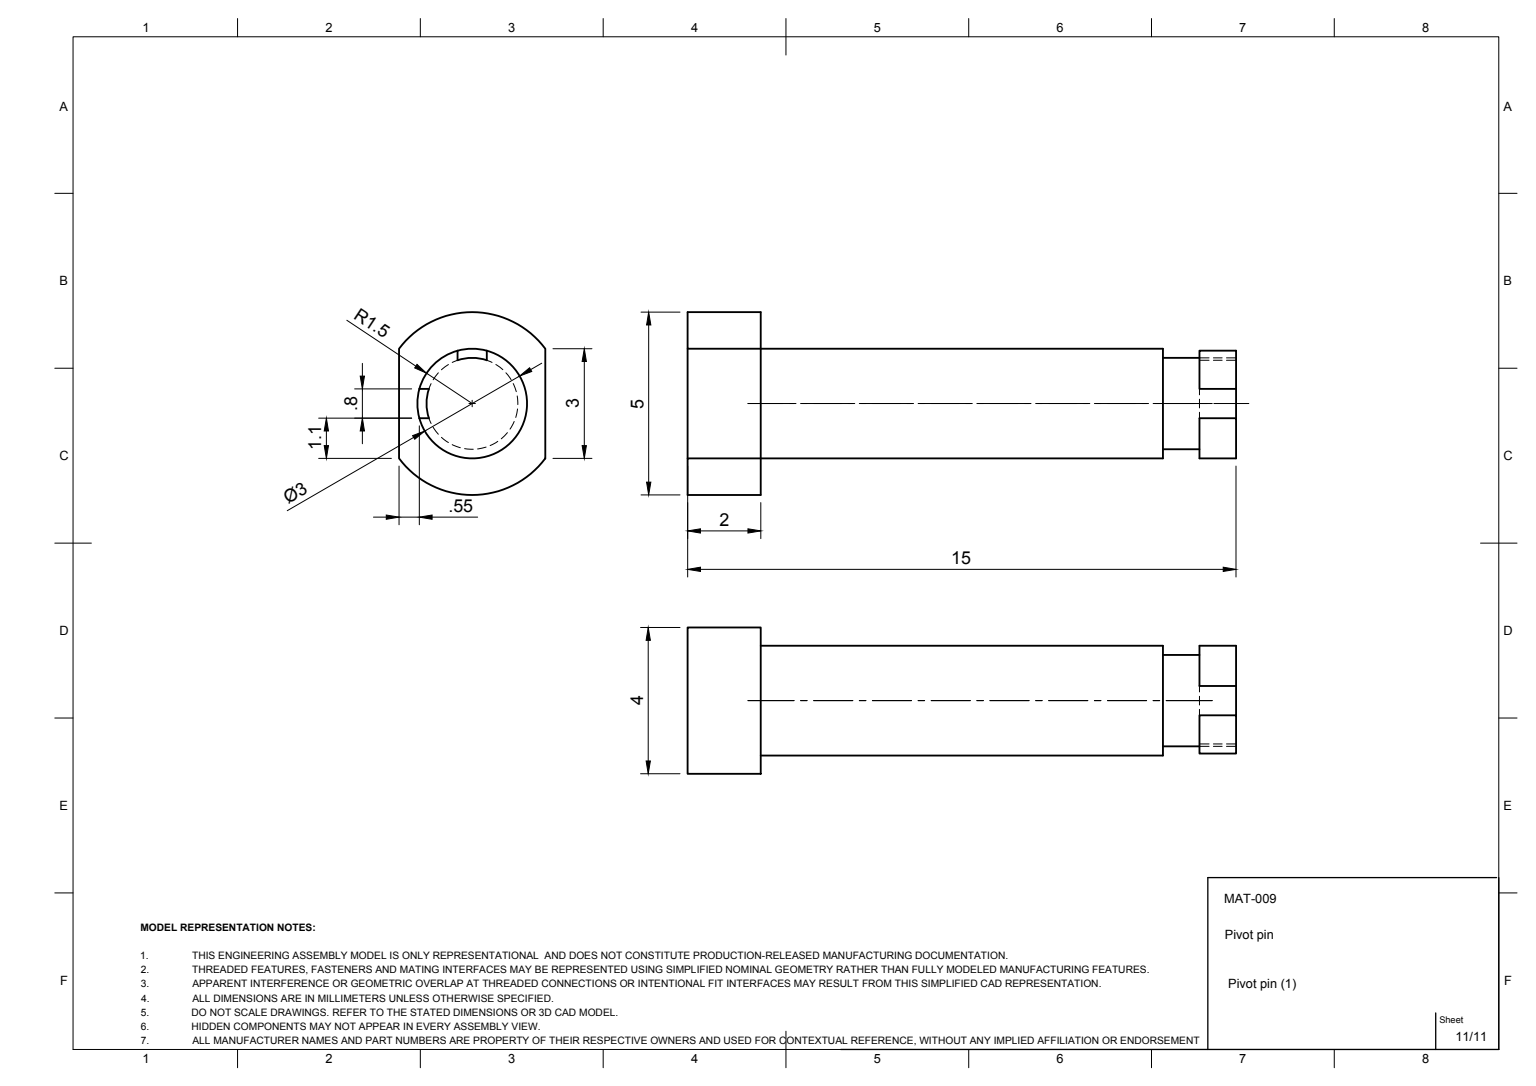
ISO-10303-21;
HEADER;
/* Generated by software containing ST-Developer
 * from STEP Tools, Inc. (www.steptools.com) 
 */

FILE_DESCRIPTION(
/* description */ ('STEP AP214'),
/* implementation_level */ '2;1');

FILE_NAME(
/* name */ 'Pivot Pin.step',
/* time_stamp */ '2026-11-14T05:43:09-08:00',
/* author */ (''),
/* organization */ (''),
/* preprocessor_version */ 'ST-DEVELOPER v20.2',
/* originating_system */ 'Autodesk Translation Framework v15.17.0.0',
/* authorisation */ '');

FILE_SCHEMA (('AUTOMOTIVE_DESIGN { 1 0 10303 214 3 1 1 }'));
ENDSEC;

DATA;
#10=MECHANICAL_DESIGN_GEOMETRIC_PRESENTATION_REPRESENTATION('',(#153),#11933);
#135=SHAPE_REPRESENTATION_RELATIONSHIP('SRR','None',#11995,#144);
#144=ADVANCED_BREP_SHAPE_REPRESENTATION('',(#162),#11931);
#153=STYLED_ITEM('',(#12043),#162);
#162=MANIFOLD_SOLID_BREP('Body1',#6650);
#206=FACE_BOUND('',#1042,.T.);
#207=FACE_BOUND('',#1051,.T.);
#298=PLANE('',#7567);
#299=PLANE('',#7571);
#300=PLANE('',#7572);
#301=PLANE('',#7576);
#302=PLANE('',#7577);
#303=PLANE('',#7578);
#304=PLANE('',#7579);
#305=PLANE('',#7580);
#306=PLANE('',#7581);
#307=PLANE('',#7586);
#308=PLANE('',#7589);
#309=PLANE('',#7590);
#641=FACE_OUTER_BOUND('',#1037,.T.);
#642=FACE_OUTER_BOUND('',#1038,.T.);
#643=FACE_OUTER_BOUND('',#1039,.T.);
#644=FACE_OUTER_BOUND('',#1040,.T.);
#645=FACE_OUTER_BOUND('',#1041,.T.);
#646=FACE_OUTER_BOUND('',#1043,.T.);
#647=FACE_OUTER_BOUND('',#1044,.T.);
#648=FACE_OUTER_BOUND('',#1045,.T.);
#649=FACE_OUTER_BOUND('',#1046,.T.);
#650=FACE_OUTER_BOUND('',#1047,.T.);
#651=FACE_OUTER_BOUND('',#1048,.T.);
#652=FACE_OUTER_BOUND('',#1049,.T.);
#653=FACE_OUTER_BOUND('',#1050,.T.);
#654=FACE_OUTER_BOUND('',#1052,.T.);
#655=FACE_OUTER_BOUND('',#1053,.T.);
#656=FACE_OUTER_BOUND('',#1054,.T.);
#657=FACE_OUTER_BOUND('',#1055,.T.);
#658=FACE_OUTER_BOUND('',#1056,.T.);
#1037=EDGE_LOOP('',(#5896,#5897,#5898,#5899,#5900,#5901,#5902,#5903,#5904,
#5905,#5906,#5907));
#1038=EDGE_LOOP('',(#5908,#5909,#5910,#5911));
#1039=EDGE_LOOP('',(#5912,#5913,#5914,#5915));
#1040=EDGE_LOOP('',(#5916,#5917,#5918,#5919));
#1041=EDGE_LOOP('',(#5920));
#1042=EDGE_LOOP('',(#5921));
#1043=EDGE_LOOP('',(#5922,#5923,#5924,#5925,#5926));
#1044=EDGE_LOOP('',(#5927,#5928,#5929,#5930));
#1045=EDGE_LOOP('',(#5931,#5932,#5933,#5934,#5935,#5936,#5937,#5938));
#1046=EDGE_LOOP('',(#5939,#5940,#5941,#5942));
#1047=EDGE_LOOP('',(#5943,#5944,#5945,#5946));
#1048=EDGE_LOOP('',(#5947,#5948,#5949,#5950));
#1049=EDGE_LOOP('',(#5951,#5952,#5953,#5954));
#1050=EDGE_LOOP('',(#5955,#5956,#5957,#5958));
#1051=EDGE_LOOP('',(#5959));
#1052=EDGE_LOOP('',(#5960,#5961,#5962,#5963));
#1053=EDGE_LOOP('',(#5964,#5965,#5966,#5967));
#1054=EDGE_LOOP('',(#5968,#5969,#5970,#5971));
#1055=EDGE_LOOP('',(#5972,#5973,#5974,#5975));
#1056=EDGE_LOOP('',(#5976,#5977,#5978,#5979));
#1490=LINE('',#11729,#1952);
#1491=LINE('',#11733,#1953);
#1492=LINE('',#11737,#1954);
#1493=LINE('',#11741,#1955);
#1494=LINE('',#11745,#1956);
#1495=LINE('',#11751,#1957);
#1496=LINE('',#11755,#1958);
#1497=LINE('',#11758,#1959);
#1498=LINE('',#11761,#1960);
#1499=LINE('',#11764,#1961);
#1500=LINE('',#11770,#1962);
#1501=LINE('',#11771,#1963);
#1502=LINE('',#11776,#1964);
#1503=LINE('',#11777,#1965);
#1504=LINE('',#11779,#1966);
#1505=LINE('',#11780,#1967);
#1506=LINE('',#11781,#1968);
#1507=LINE('',#11782,#1969);
#1508=LINE('',#11792,#1970);
#1509=LINE('',#11795,#1971);
#1510=LINE('',#11798,#1972);
#1511=LINE('',#11801,#1973);
#1512=LINE('',#11804,#1974);
#1513=LINE('',#11805,#1975);
#1514=LINE('',#11808,#1976);
#1515=LINE('',#11811,#1977);
#1952=VECTOR('',#9682,1.25);
#1953=VECTOR('',#9685,1000.);
#1954=VECTOR('',#9688,1000.);
#1955=VECTOR('',#9691,1000.);
#1956=VECTOR('',#9694,1000.);
#1957=VECTOR('',#9701,1.5);
#1958=VECTOR('',#9706,1000.);
#1959=VECTOR('',#9709,1000.);
#1960=VECTOR('',#9712,1000.);
#1961=VECTOR('',#9715,1000.);
#1962=VECTOR('',#9722,1000.);
#1963=VECTOR('',#9723,1000.);
#1964=VECTOR('',#9728,1000.);
#1965=VECTOR('',#9729,1000.);
#1966=VECTOR('',#9732,1000.);
#1967=VECTOR('',#9733,1000.);
#1968=VECTOR('',#9734,1000.);
#1969=VECTOR('',#9735,1000.);
#1970=VECTOR('',#9748,1000.);
#1971=VECTOR('',#9751,1000.);
#1972=VECTOR('',#9754,1000.);
#1973=VECTOR('',#9757,1000.);
#1974=VECTOR('',#9760,1000.);
#1975=VECTOR('',#9761,1000.);
#1976=VECTOR('',#9764,1000.);
#1977=VECTOR('',#9769,1000.);
#2470=CIRCLE('',#7558,1.25);
#2471=CIRCLE('',#7559,1.25);
#2472=CIRCLE('',#7560,1.25);
#2473=CIRCLE('',#7561,1.25);
#2474=CIRCLE('',#7562,1.25);
#2475=CIRCLE('',#7563,1.25);
#2476=CIRCLE('',#7565,1.5);
#2477=CIRCLE('',#7566,1.5);
#2478=CIRCLE('',#7568,1.5);
#2479=CIRCLE('',#7570,1.5);
#2480=CIRCLE('',#7573,1.5);
#2481=CIRCLE('',#7575,1.5);
#2482=CIRCLE('',#7582,2.5);
#2483=CIRCLE('',#7583,2.5);
#2484=CIRCLE('',#7585,2.5);
#2485=CIRCLE('',#7588,2.5);
#3095=VERTEX_POINT('',#11726);
#3096=VERTEX_POINT('',#11728);
#3097=VERTEX_POINT('',#11730);
#3098=VERTEX_POINT('',#11732);
#3099=VERTEX_POINT('',#11734);
#3100=VERTEX_POINT('',#11736);
#3101=VERTEX_POINT('',#11738);
#3102=VERTEX_POINT('',#11740);
#3103=VERTEX_POINT('',#11742);
#3104=VERTEX_POINT('',#11744);
#3105=VERTEX_POINT('',#11748);
#3106=VERTEX_POINT('',#11750);
#3107=VERTEX_POINT('',#11754);
#3108=VERTEX_POINT('',#11756);
#3109=VERTEX_POINT('',#11760);
#3110=VERTEX_POINT('',#11762);
#3111=VERTEX_POINT('',#11767);
#3112=VERTEX_POINT('',#11768);
#3113=VERTEX_POINT('',#11773);
#3114=VERTEX_POINT('',#11774);
#3115=VERTEX_POINT('',#11788);
#3116=VERTEX_POINT('',#11789);
#3117=VERTEX_POINT('',#11791);
#3118=VERTEX_POINT('',#11793);
#3119=VERTEX_POINT('',#11797);
#3120=VERTEX_POINT('',#11799);
#3121=VERTEX_POINT('',#11803);
#3122=VERTEX_POINT('',#11807);
#4037=EDGE_CURVE('',#3095,#3095,#2470,.T.);
#4038=EDGE_CURVE('',#3095,#3096,#1490,.T.);
#4039=EDGE_CURVE('',#3097,#3096,#2471,.T.);
#4040=EDGE_CURVE('',#3097,#3098,#1491,.T.);
#4041=EDGE_CURVE('',#3098,#3099,#2472,.T.);
#4042=EDGE_CURVE('',#3100,#3099,#1492,.T.);
#4043=EDGE_CURVE('',#3101,#3100,#2473,.T.);
#4044=EDGE_CURVE('',#3101,#3102,#1493,.T.);
#4045=EDGE_CURVE('',#3102,#3103,#2474,.T.);
#4046=EDGE_CURVE('',#3104,#3103,#1494,.T.);
#4047=EDGE_CURVE('',#3096,#3104,#2475,.T.);
#4048=EDGE_CURVE('',#3105,#3105,#2476,.T.);
#4049=EDGE_CURVE('',#3105,#3106,#1495,.T.);
#4050=EDGE_CURVE('',#3106,#3106,#2477,.T.);
#4051=EDGE_CURVE('',#3100,#3107,#1496,.T.);
#4052=EDGE_CURVE('',#3108,#3107,#2478,.T.);
#4053=EDGE_CURVE('',#3108,#3101,#1497,.T.);
#4054=EDGE_CURVE('',#3107,#3109,#1498,.T.);
#4055=EDGE_CURVE('',#3110,#3109,#2479,.T.);
#4056=EDGE_CURVE('',#3108,#3110,#1499,.T.);
#4057=EDGE_CURVE('',#3111,#3112,#2480,.T.);
#4058=EDGE_CURVE('',#3111,#3097,#1500,.T.);
#4059=EDGE_CURVE('',#3104,#3112,#1501,.T.);
#4060=EDGE_CURVE('',#3113,#3114,#2481,.T.);
#4061=EDGE_CURVE('',#3111,#3113,#1502,.T.);
#4062=EDGE_CURVE('',#3112,#3114,#1503,.T.);
#4063=EDGE_CURVE('',#3099,#3109,#1504,.T.);
#4064=EDGE_CURVE('',#3113,#3098,#1505,.T.);
#4065=EDGE_CURVE('',#3103,#3114,#1506,.T.);
#4066=EDGE_CURVE('',#3110,#3102,#1507,.T.);
#4067=EDGE_CURVE('',#3115,#3116,#2482,.T.);
#4068=EDGE_CURVE('',#3117,#3115,#1508,.T.);
#4069=EDGE_CURVE('',#3118,#3117,#2483,.T.);
#4070=EDGE_CURVE('',#3116,#3118,#1509,.T.);
#4071=EDGE_CURVE('',#3119,#3116,#1510,.T.);
#4072=EDGE_CURVE('',#3120,#3119,#2484,.T.);
#4073=EDGE_CURVE('',#3120,#3115,#1511,.T.);
#4074=EDGE_CURVE('',#3121,#3118,#1512,.T.);
#4075=EDGE_CURVE('',#3119,#3121,#1513,.T.);
#4076=EDGE_CURVE('',#3122,#3117,#1514,.T.);
#4077=EDGE_CURVE('',#3121,#3122,#2485,.T.);
#4078=EDGE_CURVE('',#3122,#3120,#1515,.T.);
#5896=ORIENTED_EDGE('',*,*,#4037,.T.);
#5897=ORIENTED_EDGE('',*,*,#4038,.T.);
#5898=ORIENTED_EDGE('',*,*,#4039,.F.);
#5899=ORIENTED_EDGE('',*,*,#4040,.T.);
#5900=ORIENTED_EDGE('',*,*,#4041,.T.);
#5901=ORIENTED_EDGE('',*,*,#4042,.F.);
#5902=ORIENTED_EDGE('',*,*,#4043,.F.);
#5903=ORIENTED_EDGE('',*,*,#4044,.T.);
#5904=ORIENTED_EDGE('',*,*,#4045,.T.);
#5905=ORIENTED_EDGE('',*,*,#4046,.F.);
#5906=ORIENTED_EDGE('',*,*,#4047,.F.);
#5907=ORIENTED_EDGE('',*,*,#4038,.F.);
#5908=ORIENTED_EDGE('',*,*,#4048,.F.);
#5909=ORIENTED_EDGE('',*,*,#4049,.T.);
#5910=ORIENTED_EDGE('',*,*,#4050,.F.);
#5911=ORIENTED_EDGE('',*,*,#4049,.F.);
#5912=ORIENTED_EDGE('',*,*,#4043,.T.);
#5913=ORIENTED_EDGE('',*,*,#4051,.T.);
#5914=ORIENTED_EDGE('',*,*,#4052,.F.);
#5915=ORIENTED_EDGE('',*,*,#4053,.T.);
#5916=ORIENTED_EDGE('',*,*,#4052,.T.);
#5917=ORIENTED_EDGE('',*,*,#4054,.T.);
#5918=ORIENTED_EDGE('',*,*,#4055,.F.);
#5919=ORIENTED_EDGE('',*,*,#4056,.F.);
#5920=ORIENTED_EDGE('',*,*,#4050,.T.);
#5921=ORIENTED_EDGE('',*,*,#4037,.F.);
#5922=ORIENTED_EDGE('',*,*,#4057,.F.);
#5923=ORIENTED_EDGE('',*,*,#4058,.T.);
#5924=ORIENTED_EDGE('',*,*,#4039,.T.);
#5925=ORIENTED_EDGE('',*,*,#4047,.T.);
#5926=ORIENTED_EDGE('',*,*,#4059,.T.);
#5927=ORIENTED_EDGE('',*,*,#4060,.F.);
#5928=ORIENTED_EDGE('',*,*,#4061,.F.);
#5929=ORIENTED_EDGE('',*,*,#4057,.T.);
#5930=ORIENTED_EDGE('',*,*,#4062,.T.);
#5931=ORIENTED_EDGE('',*,*,#4063,.F.);
#5932=ORIENTED_EDGE('',*,*,#4041,.F.);
#5933=ORIENTED_EDGE('',*,*,#4064,.F.);
#5934=ORIENTED_EDGE('',*,*,#4060,.T.);
#5935=ORIENTED_EDGE('',*,*,#4065,.F.);
#5936=ORIENTED_EDGE('',*,*,#4045,.F.);
#5937=ORIENTED_EDGE('',*,*,#4066,.F.);
#5938=ORIENTED_EDGE('',*,*,#4055,.T.);
#5939=ORIENTED_EDGE('',*,*,#4065,.T.);
#5940=ORIENTED_EDGE('',*,*,#4062,.F.);
#5941=ORIENTED_EDGE('',*,*,#4059,.F.);
#5942=ORIENTED_EDGE('',*,*,#4046,.T.);
#5943=ORIENTED_EDGE('',*,*,#4066,.T.);
#5944=ORIENTED_EDGE('',*,*,#4044,.F.);
#5945=ORIENTED_EDGE('',*,*,#4053,.F.);
#5946=ORIENTED_EDGE('',*,*,#4056,.T.);
#5947=ORIENTED_EDGE('',*,*,#4063,.T.);
#5948=ORIENTED_EDGE('',*,*,#4054,.F.);
#5949=ORIENTED_EDGE('',*,*,#4051,.F.);
#5950=ORIENTED_EDGE('',*,*,#4042,.T.);
#5951=ORIENTED_EDGE('',*,*,#4064,.T.);
#5952=ORIENTED_EDGE('',*,*,#4040,.F.);
#5953=ORIENTED_EDGE('',*,*,#4058,.F.);
#5954=ORIENTED_EDGE('',*,*,#4061,.T.);
#5955=ORIENTED_EDGE('',*,*,#4067,.F.);
#5956=ORIENTED_EDGE('',*,*,#4068,.F.);
#5957=ORIENTED_EDGE('',*,*,#4069,.F.);
#5958=ORIENTED_EDGE('',*,*,#4070,.F.);
#5959=ORIENTED_EDGE('',*,*,#4048,.T.);
#5960=ORIENTED_EDGE('',*,*,#4067,.T.);
#5961=ORIENTED_EDGE('',*,*,#4071,.F.);
#5962=ORIENTED_EDGE('',*,*,#4072,.F.);
#5963=ORIENTED_EDGE('',*,*,#4073,.T.);
#5964=ORIENTED_EDGE('',*,*,#4070,.T.);
#5965=ORIENTED_EDGE('',*,*,#4074,.F.);
#5966=ORIENTED_EDGE('',*,*,#4075,.F.);
#5967=ORIENTED_EDGE('',*,*,#4071,.T.);
#5968=ORIENTED_EDGE('',*,*,#4069,.T.);
#5969=ORIENTED_EDGE('',*,*,#4076,.F.);
#5970=ORIENTED_EDGE('',*,*,#4077,.F.);
#5971=ORIENTED_EDGE('',*,*,#4074,.T.);
#5972=ORIENTED_EDGE('',*,*,#4068,.T.);
#5973=ORIENTED_EDGE('',*,*,#4073,.F.);
#5974=ORIENTED_EDGE('',*,*,#4078,.F.);
#5975=ORIENTED_EDGE('',*,*,#4076,.T.);
#5976=ORIENTED_EDGE('',*,*,#4072,.T.);
#5977=ORIENTED_EDGE('',*,*,#4075,.T.);
#5978=ORIENTED_EDGE('',*,*,#4077,.T.);
#5979=ORIENTED_EDGE('',*,*,#4078,.T.);
#6279=CYLINDRICAL_SURFACE('',#7557,1.25);
#6280=CYLINDRICAL_SURFACE('',#7564,1.5);
#6281=CYLINDRICAL_SURFACE('',#7569,1.5);
#6282=CYLINDRICAL_SURFACE('',#7574,1.5);
#6283=CYLINDRICAL_SURFACE('',#7584,2.5);
#6284=CYLINDRICAL_SURFACE('',#7587,2.5);
#6611=ADVANCED_FACE('',(#641),#6279,.T.);
#6612=ADVANCED_FACE('',(#642),#6280,.T.);
#6613=ADVANCED_FACE('',(#643),#298,.F.);
#6614=ADVANCED_FACE('',(#644),#6281,.T.);
#6615=ADVANCED_FACE('',(#645,#206),#299,.T.);
#6616=ADVANCED_FACE('',(#646),#300,.F.);
#6617=ADVANCED_FACE('',(#647),#6282,.T.);
#6618=ADVANCED_FACE('',(#648),#301,.T.);
#6619=ADVANCED_FACE('',(#649),#302,.F.);
#6620=ADVANCED_FACE('',(#650),#303,.F.);
#6621=ADVANCED_FACE('',(#651),#304,.F.);
#6622=ADVANCED_FACE('',(#652),#305,.F.);
#6623=ADVANCED_FACE('',(#653,#207),#306,.F.);
#6624=ADVANCED_FACE('',(#654),#6283,.T.);
#6625=ADVANCED_FACE('',(#655),#307,.F.);
#6626=ADVANCED_FACE('',(#656),#6284,.T.);
#6627=ADVANCED_FACE('',(#657),#308,.F.);
#6628=ADVANCED_FACE('',(#658),#309,.T.);
#6650=CLOSED_SHELL('',(#6611,#6612,#6613,#6614,#6615,#6616,#6617,#6618,
#6619,#6620,#6621,#6622,#6623,#6624,#6625,#6626,#6627,#6628));
#7556=AXIS2_PLACEMENT_3D('',#11724,#9676,#9677);
#7557=AXIS2_PLACEMENT_3D('',#11725,#9678,#9679);
#7558=AXIS2_PLACEMENT_3D('',#11727,#9680,#9681);
#7559=AXIS2_PLACEMENT_3D('',#11731,#9683,#9684);
#7560=AXIS2_PLACEMENT_3D('',#11735,#9686,#9687);
#7561=AXIS2_PLACEMENT_3D('',#11739,#9689,#9690);
#7562=AXIS2_PLACEMENT_3D('',#11743,#9692,#9693);
#7563=AXIS2_PLACEMENT_3D('',#11746,#9695,#9696);
#7564=AXIS2_PLACEMENT_3D('',#11747,#9697,#9698);
#7565=AXIS2_PLACEMENT_3D('',#11749,#9699,#9700);
#7566=AXIS2_PLACEMENT_3D('',#11752,#9702,#9703);
#7567=AXIS2_PLACEMENT_3D('',#11753,#9704,#9705);
#7568=AXIS2_PLACEMENT_3D('',#11757,#9707,#9708);
#7569=AXIS2_PLACEMENT_3D('',#11759,#9710,#9711);
#7570=AXIS2_PLACEMENT_3D('',#11763,#9713,#9714);
#7571=AXIS2_PLACEMENT_3D('',#11765,#9716,#9717);
#7572=AXIS2_PLACEMENT_3D('',#11766,#9718,#9719);
#7573=AXIS2_PLACEMENT_3D('',#11769,#9720,#9721);
#7574=AXIS2_PLACEMENT_3D('',#11772,#9724,#9725);
#7575=AXIS2_PLACEMENT_3D('',#11775,#9726,#9727);
#7576=AXIS2_PLACEMENT_3D('',#11778,#9730,#9731);
#7577=AXIS2_PLACEMENT_3D('',#11783,#9736,#9737);
#7578=AXIS2_PLACEMENT_3D('',#11784,#9738,#9739);
#7579=AXIS2_PLACEMENT_3D('',#11785,#9740,#9741);
#7580=AXIS2_PLACEMENT_3D('',#11786,#9742,#9743);
#7581=AXIS2_PLACEMENT_3D('',#11787,#9744,#9745);
#7582=AXIS2_PLACEMENT_3D('',#11790,#9746,#9747);
#7583=AXIS2_PLACEMENT_3D('',#11794,#9749,#9750);
#7584=AXIS2_PLACEMENT_3D('',#11796,#9752,#9753);
#7585=AXIS2_PLACEMENT_3D('',#11800,#9755,#9756);
#7586=AXIS2_PLACEMENT_3D('',#11802,#9758,#9759);
#7587=AXIS2_PLACEMENT_3D('',#11806,#9762,#9763);
#7588=AXIS2_PLACEMENT_3D('',#11809,#9765,#9766);
#7589=AXIS2_PLACEMENT_3D('',#11810,#9767,#9768);
#7590=AXIS2_PLACEMENT_3D('',#11812,#9770,#9771);
#9676=DIRECTION('axis',(0.,0.,1.));
#9677=DIRECTION('refdir',(1.,0.,0.));
#9678=DIRECTION('center_axis',(0.,0.,-1.));
#9679=DIRECTION('ref_axis',(-1.,0.,0.));
#9680=DIRECTION('center_axis',(0.,0.,1.));
#9681=DIRECTION('ref_axis',(1.,0.,0.));
#9682=DIRECTION('',(0.,0.,1.));
#9683=DIRECTION('center_axis',(0.,0.,1.));
#9684=DIRECTION('ref_axis',(1.,0.,0.));
#9685=DIRECTION('',(0.,0.,1.));
#9686=DIRECTION('center_axis',(0.,0.,-1.));
#9687=DIRECTION('ref_axis',(1.,0.,0.));
#9688=DIRECTION('',(0.,0.,1.));
#9689=DIRECTION('center_axis',(0.,0.,1.));
#9690=DIRECTION('ref_axis',(1.,0.,0.));
#9691=DIRECTION('',(0.,0.,1.));
#9692=DIRECTION('center_axis',(0.,0.,-1.));
#9693=DIRECTION('ref_axis',(1.,0.,0.));
#9694=DIRECTION('',(0.,0.,1.));
#9695=DIRECTION('center_axis',(0.,0.,1.));
#9696=DIRECTION('ref_axis',(1.,0.,0.));
#9697=DIRECTION('center_axis',(0.,0.,-1.));
#9698=DIRECTION('ref_axis',(-1.,0.,0.));
#9699=DIRECTION('center_axis',(0.,0.,-1.));
#9700=DIRECTION('ref_axis',(-1.,0.,0.));
#9701=DIRECTION('',(0.,0.,1.));
#9702=DIRECTION('center_axis',(0.,0.,1.));
#9703=DIRECTION('ref_axis',(1.,0.,0.));
#9704=DIRECTION('center_axis',(0.,0.,1.));
#9705=DIRECTION('ref_axis',(1.,0.,0.));
#9706=DIRECTION('',(-1.,2.07374770584121E-16,0.));
#9707=DIRECTION('center_axis',(0.,0.,1.));
#9708=DIRECTION('ref_axis',(1.,0.,0.));
#9709=DIRECTION('',(2.07374770584121E-16,-1.,0.));
#9710=DIRECTION('center_axis',(0.,0.,-1.));
#9711=DIRECTION('ref_axis',(-1.,0.,0.));
#9712=DIRECTION('',(0.,0.,1.));
#9713=DIRECTION('center_axis',(0.,0.,1.));
#9714=DIRECTION('ref_axis',(1.,0.,0.));
#9715=DIRECTION('',(0.,0.,1.));
#9716=DIRECTION('center_axis',(0.,0.,1.));
#9717=DIRECTION('ref_axis',(1.,0.,0.));
#9718=DIRECTION('center_axis',(0.,0.,1.));
#9719=DIRECTION('ref_axis',(1.,0.,0.));
#9720=DIRECTION('center_axis',(0.,0.,1.));
#9721=DIRECTION('ref_axis',(1.,0.,0.));
#9722=DIRECTION('',(1.,2.07374770584121E-16,0.));
#9723=DIRECTION('',(2.07374770584121E-16,1.,0.));
#9724=DIRECTION('center_axis',(0.,0.,-1.));
#9725=DIRECTION('ref_axis',(0.707106781186548,-0.707106781186547,0.));
#9726=DIRECTION('center_axis',(0.,0.,1.));
#9727=DIRECTION('ref_axis',(1.,0.,0.));
#9728=DIRECTION('',(0.,0.,1.));
#9729=DIRECTION('',(0.,0.,1.));
#9730=DIRECTION('center_axis',(0.,0.,1.));
#9731=DIRECTION('ref_axis',(1.,0.,0.));
#9732=DIRECTION('',(-1.,2.07374770584121E-16,0.));
#9733=DIRECTION('',(1.,2.07374770584121E-16,0.));
#9734=DIRECTION('',(2.07374770584121E-16,1.,0.));
#9735=DIRECTION('',(2.07374770584121E-16,-1.,0.));
#9736=DIRECTION('center_axis',(1.,-2.07374770584121E-16,0.));
#9737=DIRECTION('ref_axis',(2.07374770584121E-16,1.,0.));
#9738=DIRECTION('center_axis',(-1.,-2.07374770584121E-16,0.));
#9739=DIRECTION('ref_axis',(2.07374770584121E-16,-1.,0.));
#9740=DIRECTION('center_axis',(2.07374770584121E-16,1.,0.));
#9741=DIRECTION('ref_axis',(-1.,2.07374770584121E-16,0.));
#9742=DIRECTION('center_axis',(2.07374770584121E-16,-1.,0.));
#9743=DIRECTION('ref_axis',(1.,2.07374770584121E-16,0.));
#9744=DIRECTION('center_axis',(0.,0.,-1.));
#9745=DIRECTION('ref_axis',(-1.,0.,0.));
#9746=DIRECTION('center_axis',(0.,0.,-1.));
#9747=DIRECTION('ref_axis',(-1.,0.,0.));
#9748=DIRECTION('',(0.,1.,0.));
#9749=DIRECTION('center_axis',(0.,0.,-1.));
#9750=DIRECTION('ref_axis',(-1.,0.,0.));
#9751=DIRECTION('',(0.,-1.,0.));
#9752=DIRECTION('center_axis',(0.,0.,1.));
#9753=DIRECTION('ref_axis',(1.,0.,0.));
#9754=DIRECTION('',(0.,0.,1.));
#9755=DIRECTION('center_axis',(0.,0.,-1.));
#9756=DIRECTION('ref_axis',(-1.,0.,0.));
#9757=DIRECTION('',(0.,0.,1.));
#9758=DIRECTION('center_axis',(-1.,0.,0.));
#9759=DIRECTION('ref_axis',(0.,0.,1.));
#9760=DIRECTION('',(0.,0.,1.));
#9761=DIRECTION('',(0.,-1.,0.));
#9762=DIRECTION('center_axis',(0.,0.,1.));
#9763=DIRECTION('ref_axis',(1.,0.,0.));
#9764=DIRECTION('',(0.,0.,1.));
#9765=DIRECTION('center_axis',(0.,0.,-1.));
#9766=DIRECTION('ref_axis',(-1.,0.,0.));
#9767=DIRECTION('center_axis',(1.,0.,0.));
#9768=DIRECTION('ref_axis',(0.,0.,-1.));
#9769=DIRECTION('',(0.,1.,0.));
#9770=DIRECTION('center_axis',(0.,0.,-1.));
#9771=DIRECTION('ref_axis',(-1.,0.,0.));
#11724=CARTESIAN_POINT('',(0.,0.,0.));
#11725=CARTESIAN_POINT('Origin',(0.,0.,16.));
#11726=CARTESIAN_POINT('',(1.25,-1.53080849893419E-16,15.));
#11727=CARTESIAN_POINT('Origin',(0.,0.,15.));
#11728=CARTESIAN_POINT('',(1.25,-1.53080849893419E-16,16.));
#11729=CARTESIAN_POINT('',(1.25,-1.53080849893419E-16,16.));
#11730=CARTESIAN_POINT('',(-1.1842719282327,-0.4,16.));
#11731=CARTESIAN_POINT('Origin',(0.,0.,16.));
#11732=CARTESIAN_POINT('',(-1.1842719282327,-0.4,17.));
#11733=CARTESIAN_POINT('',(-1.1842719282327,-0.4,16.));
#11734=CARTESIAN_POINT('',(-1.1842719282327,0.4,17.));
#11735=CARTESIAN_POINT('Origin',(0.,0.,17.));
#11736=CARTESIAN_POINT('',(-1.1842719282327,0.4,16.));
#11737=CARTESIAN_POINT('',(-1.1842719282327,0.4,16.));
#11738=CARTESIAN_POINT('',(-0.4,1.1842719282327,16.));
#11739=CARTESIAN_POINT('Origin',(0.,0.,16.));
#11740=CARTESIAN_POINT('',(-0.4,1.1842719282327,17.));
#11741=CARTESIAN_POINT('',(-0.4,1.1842719282327,16.));
#11742=CARTESIAN_POINT('',(0.4,1.1842719282327,17.));
#11743=CARTESIAN_POINT('Origin',(0.,0.,17.));
#11744=CARTESIAN_POINT('',(0.4,1.1842719282327,16.));
#11745=CARTESIAN_POINT('',(0.4,1.1842719282327,16.));
#11746=CARTESIAN_POINT('Origin',(0.,0.,16.));
#11747=CARTESIAN_POINT('Origin',(0.,0.,15.));
#11748=CARTESIAN_POINT('',(1.5,-1.83697019872103E-16,4.));
#11749=CARTESIAN_POINT('Origin',(0.,0.,4.));
#11750=CARTESIAN_POINT('',(1.5,-1.83697019872103E-16,15.));
#11751=CARTESIAN_POINT('',(1.5,-1.83697019872103E-16,15.));
#11752=CARTESIAN_POINT('Origin',(0.,0.,15.));
#11753=CARTESIAN_POINT('Origin',(0.,0.,16.));
#11754=CARTESIAN_POINT('',(-1.4456832294801,0.4,16.));
#11755=CARTESIAN_POINT('',(-1.1842719282327,0.4,16.));
#11756=CARTESIAN_POINT('',(-0.4,1.4456832294801,16.));
#11757=CARTESIAN_POINT('Origin',(0.,0.,16.));
#11758=CARTESIAN_POINT('',(-0.4,1.1842719282327,16.));
#11759=CARTESIAN_POINT('Origin',(0.,0.,17.));
#11760=CARTESIAN_POINT('',(-1.4456832294801,0.4,17.));
#11761=CARTESIAN_POINT('',(-1.4456832294801,0.4,16.));
#11762=CARTESIAN_POINT('',(-0.4,1.4456832294801,17.));
#11763=CARTESIAN_POINT('Origin',(0.,0.,17.));
#11764=CARTESIAN_POINT('',(-0.4,1.4456832294801,16.));
#11765=CARTESIAN_POINT('Origin',(0.,0.,15.));
#11766=CARTESIAN_POINT('Origin',(0.,0.,16.));
#11767=CARTESIAN_POINT('',(-1.4456832294801,-0.4,16.));
#11768=CARTESIAN_POINT('',(0.4,1.4456832294801,16.));
#11769=CARTESIAN_POINT('Origin',(0.,0.,16.));
#11770=CARTESIAN_POINT('',(-1.1842719282327,-0.4,16.));
#11771=CARTESIAN_POINT('',(0.4,1.1842719282327,16.));
#11772=CARTESIAN_POINT('Origin',(0.,0.,17.));
#11773=CARTESIAN_POINT('',(-1.4456832294801,-0.4,17.));
#11774=CARTESIAN_POINT('',(0.4,1.4456832294801,17.));
#11775=CARTESIAN_POINT('Origin',(0.,0.,17.));
#11776=CARTESIAN_POINT('',(-1.4456832294801,-0.4,16.));
#11777=CARTESIAN_POINT('',(0.4,1.4456832294801,16.));
#11778=CARTESIAN_POINT('Origin',(0.,0.,17.));
#11779=CARTESIAN_POINT('',(-1.1842719282327,0.4,17.));
#11780=CARTESIAN_POINT('',(-1.1842719282327,-0.4,17.));
#11781=CARTESIAN_POINT('',(0.4,1.1842719282327,17.));
#11782=CARTESIAN_POINT('',(-0.4,1.1842719282327,17.));
#11783=CARTESIAN_POINT('Origin',(0.4,1.1842719282327,16.));
#11784=CARTESIAN_POINT('Origin',(-0.4,1.1842719282327,16.));
#11785=CARTESIAN_POINT('Origin',(-1.1842719282327,0.4,16.));
#11786=CARTESIAN_POINT('Origin',(-1.1842719282327,-0.4,16.));
#11787=CARTESIAN_POINT('Origin',(0.,0.,4.));
#11788=CARTESIAN_POINT('',(-2.,1.5,4.));
#11789=CARTESIAN_POINT('',(2.,1.5,4.));
#11790=CARTESIAN_POINT('Origin',(0.,0.,4.));
#11791=CARTESIAN_POINT('',(-2.,-1.5,4.));
#11792=CARTESIAN_POINT('',(-2.,1.5,4.));
#11793=CARTESIAN_POINT('',(2.,-1.5,4.));
#11794=CARTESIAN_POINT('Origin',(0.,0.,4.));
#11795=CARTESIAN_POINT('',(2.,1.5,4.));
#11796=CARTESIAN_POINT('Origin',(0.,0.,2.));
#11797=CARTESIAN_POINT('',(2.,1.5,2.));
#11798=CARTESIAN_POINT('',(2.,1.5,2.));
#11799=CARTESIAN_POINT('',(-2.,1.5,2.));
#11800=CARTESIAN_POINT('Origin',(0.,0.,2.));
#11801=CARTESIAN_POINT('',(-2.,1.5,2.));
#11802=CARTESIAN_POINT('Origin',(2.,1.5,2.));
#11803=CARTESIAN_POINT('',(2.,-1.5,2.));
#11804=CARTESIAN_POINT('',(2.,-1.5,2.));
#11805=CARTESIAN_POINT('',(2.,1.5,2.));
#11806=CARTESIAN_POINT('Origin',(0.,0.,2.));
#11807=CARTESIAN_POINT('',(-2.,-1.5,2.));
#11808=CARTESIAN_POINT('',(-2.,-1.5,2.));
#11809=CARTESIAN_POINT('Origin',(0.,0.,2.));
#11810=CARTESIAN_POINT('Origin',(-2.,1.5,2.));
#11811=CARTESIAN_POINT('',(-2.,1.5,2.));
#11812=CARTESIAN_POINT('Origin',(0.,0.,2.));
#11920=UNCERTAINTY_MEASURE_WITH_UNIT(LENGTH_MEASURE(0.01),#11934,
'DISTANCE_ACCURACY_VALUE',
'Maximum model space distance between geometric entities at asserted c
onnectivities');
#11922=UNCERTAINTY_MEASURE_WITH_UNIT(LENGTH_MEASURE(0.01),#11934,
'DISTANCE_ACCURACY_VALUE',
'Maximum model space distance between geometric entities at asserted c
onnectivities');
#11931=(
GEOMETRIC_REPRESENTATION_CONTEXT(3)
GLOBAL_UNCERTAINTY_ASSIGNED_CONTEXT((#11920))
GLOBAL_UNIT_ASSIGNED_CONTEXT((#11934,#11936,#11937))
REPRESENTATION_CONTEXT('','3D')
);
#11933=(
GEOMETRIC_REPRESENTATION_CONTEXT(3)
GLOBAL_UNCERTAINTY_ASSIGNED_CONTEXT((#11922))
GLOBAL_UNIT_ASSIGNED_CONTEXT((#11934,#11936,#11937))
REPRESENTATION_CONTEXT('','3D')
);
#11934=(
LENGTH_UNIT()
NAMED_UNIT(*)
SI_UNIT(.MILLI.,.METRE.)
);
#11936=(
NAMED_UNIT(*)
PLANE_ANGLE_UNIT()
SI_UNIT($,.RADIAN.)
);
#11937=(
NAMED_UNIT(*)
SI_UNIT($,.STERADIAN.)
SOLID_ANGLE_UNIT()
);
#11946=SHAPE_DEFINITION_REPRESENTATION(#11956,#11995);
#11956=PRODUCT_DEFINITION_SHAPE('',$,#12006);
#11995=SHAPE_REPRESENTATION('',(#7556),#11931);
#11997=PRODUCT_DEFINITION_CONTEXT('part definition',#12029,'design');
#12006=PRODUCT_DEFINITION('Pivot pin','Pivot Pin',#12016,#11997);
#12016=PRODUCT_DEFINITION_FORMATION('',$,#12039);
#12029=APPLICATION_CONTEXT(
'Core Data for Automotive Mechanical Design Process');
#12030=PRODUCT_CONTEXT('part definition',#12029,'mechanical');
#12039=PRODUCT('Pivot pin','Pivot Pin','Pivot pin',(#12030));
#12043=PRESENTATION_STYLE_ASSIGNMENT((#12047));
#12047=SURFACE_STYLE_USAGE(.BOTH.,#12051);
#12051=SURFACE_SIDE_STYLE('',(#12055));
#12055=SURFACE_STYLE_FILL_AREA(#12059);
#12059=FILL_AREA_STYLE('Opaque(61,176,222)',(#12063));
#12063=FILL_AREA_STYLE_COLOUR('Opaque(61,176,222)',#12067);
#12067=COLOUR_RGB('Opaque(61,176,222)',0.23921568627451,0.690196078431373,
0.870588235294118);
ENDSEC;
END-ISO-10303-21;
